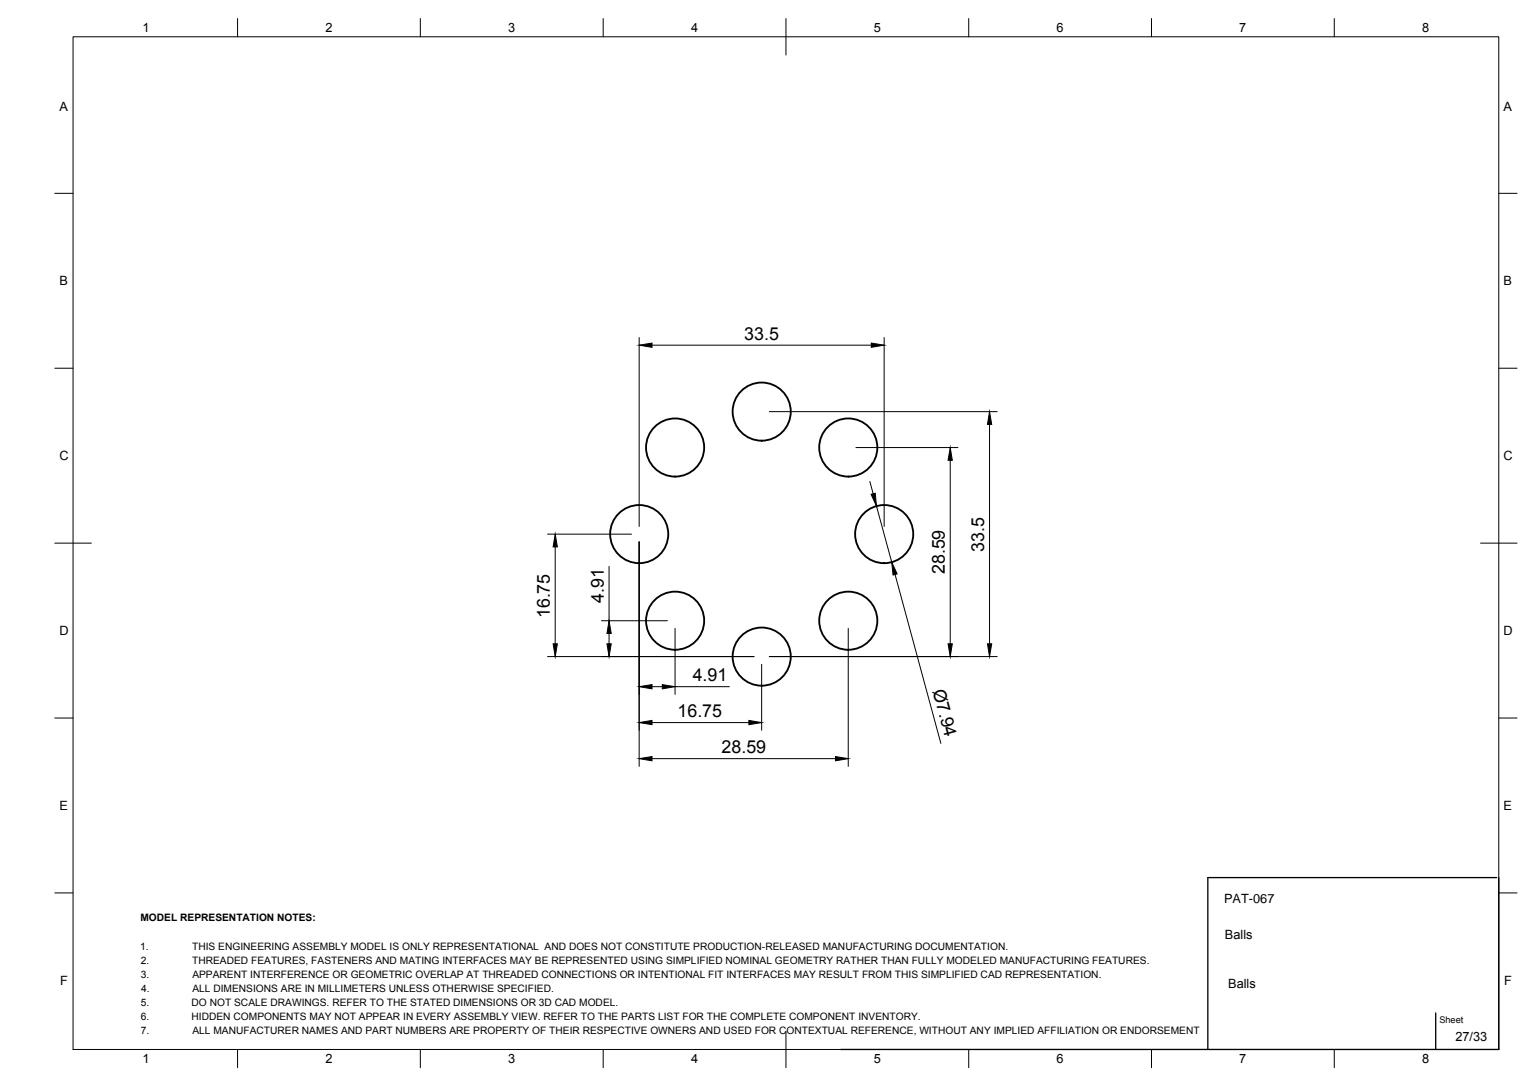
ISO-10303-21;
HEADER;
/* Generated by software containing ST-Developer
 * from STEP Tools, Inc. (www.steptools.com) 
 */

FILE_DESCRIPTION(
/* description */ ('Lifting hook block with sheave'),
/* implementation_level */ '2;1');

FILE_NAME(
/* name */ 'Balls.step',
/* time_stamp */ '2026-10-28T03:23:54-07:00',
/* author */ (''),
/* organization */ (''),
/* preprocessor_version */ 'ST-DEVELOPER v20.2',
/* originating_system */ 'Autodesk Translation Framework v15.17.0.0',
/* authorisation */ '');

FILE_SCHEMA (('AUTOMOTIVE_DESIGN { 1 0 10303 214 3 1 1 }'));
ENDSEC;

DATA;
#10=MECHANICAL_DESIGN_GEOMETRIC_PRESENTATION_REPRESENTATION('',(#373,#374,#375,#376,#377,#378,#379,#380),#9391);
#29=SPHERICAL_SURFACE('',#5724,0.3969);
#30=SPHERICAL_SURFACE('',#5726,0.3969);
#31=SPHERICAL_SURFACE('',#5728,0.3969);
#32=SPHERICAL_SURFACE('',#5730,0.3969);
#33=SPHERICAL_SURFACE('',#5732,0.3969);
#34=SPHERICAL_SURFACE('',#5734,0.3969);
#35=SPHERICAL_SURFACE('',#5736,0.3969);
#36=SPHERICAL_SURFACE('',#5738,0.3969);
#313=SHAPE_REPRESENTATION_RELATIONSHIP('SRR','None',#9546,#343);
#343=ADVANCED_BREP_SHAPE_REPRESENTATION('',(#409,#410,#411,#412,#413,#414,
#415,#416),#9381);
#373=STYLED_ITEM('',(#9759),#409);
#374=STYLED_ITEM('',(#9759),#410);
#375=STYLED_ITEM('',(#9759),#411);
#376=STYLED_ITEM('',(#9759),#412);
#377=STYLED_ITEM('',(#9759),#413);
#378=STYLED_ITEM('',(#9759),#414);
#379=STYLED_ITEM('',(#9759),#415);
#380=STYLED_ITEM('',(#9759),#416);
#409=MANIFOLD_SOLID_BREP('Body1',#4911);
#410=MANIFOLD_SOLID_BREP('Body2',#4912);
#411=MANIFOLD_SOLID_BREP('Body3',#4913);
#412=MANIFOLD_SOLID_BREP('Body4',#4914);
#413=MANIFOLD_SOLID_BREP('Body5',#4915);
#414=MANIFOLD_SOLID_BREP('Body6',#4916);
#415=MANIFOLD_SOLID_BREP('Body7',#4917);
#416=MANIFOLD_SOLID_BREP('Body8',#4918);
#1425=FACE_OUTER_BOUND('',#1813,.T.);
#1426=FACE_OUTER_BOUND('',#1814,.T.);
#1427=FACE_OUTER_BOUND('',#1815,.T.);
#1428=FACE_OUTER_BOUND('',#1816,.T.);
#1429=FACE_OUTER_BOUND('',#1817,.T.);
#1430=FACE_OUTER_BOUND('',#1818,.T.);
#1431=FACE_OUTER_BOUND('',#1819,.T.);
#1432=FACE_OUTER_BOUND('',#1820,.T.);
#1813=EDGE_LOOP('',(#4098,#4099));
#1814=EDGE_LOOP('',(#4100,#4101));
#1815=EDGE_LOOP('',(#4102,#4103));
#1816=EDGE_LOOP('',(#4104,#4105));
#1817=EDGE_LOOP('',(#4106,#4107));
#1818=EDGE_LOOP('',(#4108,#4109));
#1819=EDGE_LOOP('',(#4110,#4111));
#1820=EDGE_LOOP('',(#4112,#4113));
#2125=CIRCLE('',#5725,0.3969);
#2126=CIRCLE('',#5727,0.3969);
#2127=CIRCLE('',#5729,0.3969);
#2128=CIRCLE('',#5731,0.3969);
#2129=CIRCLE('',#5733,0.3969);
#2130=CIRCLE('',#5735,0.3969);
#2131=CIRCLE('',#5737,0.3969);
#2132=CIRCLE('',#5739,0.3969);
#2492=VERTEX_POINT('',#8555);
#2493=VERTEX_POINT('',#8556);
#2494=VERTEX_POINT('',#8559);
#2495=VERTEX_POINT('',#8560);
#2496=VERTEX_POINT('',#8563);
#2497=VERTEX_POINT('',#8564);
#2498=VERTEX_POINT('',#8567);
#2499=VERTEX_POINT('',#8568);
#2500=VERTEX_POINT('',#8571);
#2501=VERTEX_POINT('',#8572);
#2502=VERTEX_POINT('',#8575);
#2503=VERTEX_POINT('',#8576);
#2504=VERTEX_POINT('',#8579);
#2505=VERTEX_POINT('',#8580);
#2506=VERTEX_POINT('',#8583);
#2507=VERTEX_POINT('',#8584);
#3053=EDGE_CURVE('',#2492,#2493,#2125,.T.);
#3054=EDGE_CURVE('',#2494,#2495,#2126,.T.);
#3055=EDGE_CURVE('',#2496,#2497,#2127,.T.);
#3056=EDGE_CURVE('',#2498,#2499,#2128,.T.);
#3057=EDGE_CURVE('',#2500,#2501,#2129,.T.);
#3058=EDGE_CURVE('',#2502,#2503,#2130,.T.);
#3059=EDGE_CURVE('',#2504,#2505,#2131,.T.);
#3060=EDGE_CURVE('',#2506,#2507,#2132,.T.);
#4098=ORIENTED_EDGE('',*,*,#3053,.T.);
#4099=ORIENTED_EDGE('',*,*,#3053,.F.);
#4100=ORIENTED_EDGE('',*,*,#3054,.T.);
#4101=ORIENTED_EDGE('',*,*,#3054,.F.);
#4102=ORIENTED_EDGE('',*,*,#3055,.T.);
#4103=ORIENTED_EDGE('',*,*,#3055,.F.);
#4104=ORIENTED_EDGE('',*,*,#3056,.T.);
#4105=ORIENTED_EDGE('',*,*,#3056,.F.);
#4106=ORIENTED_EDGE('',*,*,#3057,.T.);
#4107=ORIENTED_EDGE('',*,*,#3057,.F.);
#4108=ORIENTED_EDGE('',*,*,#3058,.T.);
#4109=ORIENTED_EDGE('',*,*,#3058,.F.);
#4110=ORIENTED_EDGE('',*,*,#3059,.T.);
#4111=ORIENTED_EDGE('',*,*,#3059,.F.);
#4112=ORIENTED_EDGE('',*,*,#3060,.T.);
#4113=ORIENTED_EDGE('',*,*,#3060,.F.);
#4801=ADVANCED_FACE('',(#1425),#29,.T.);
#4802=ADVANCED_FACE('',(#1426),#30,.T.);
#4803=ADVANCED_FACE('',(#1427),#31,.T.);
#4804=ADVANCED_FACE('',(#1428),#32,.T.);
#4805=ADVANCED_FACE('',(#1429),#33,.T.);
#4806=ADVANCED_FACE('',(#1430),#34,.T.);
#4807=ADVANCED_FACE('',(#1431),#35,.T.);
#4808=ADVANCED_FACE('',(#1432),#36,.T.);
#4911=CLOSED_SHELL('',(#4801));
#4912=CLOSED_SHELL('',(#4802));
#4913=CLOSED_SHELL('',(#4803));
#4914=CLOSED_SHELL('',(#4804));
#4915=CLOSED_SHELL('',(#4805));
#4916=CLOSED_SHELL('',(#4806));
#4917=CLOSED_SHELL('',(#4807));
#4918=CLOSED_SHELL('',(#4808));
#5723=AXIS2_PLACEMENT_3D('',#8553,#7069,#7070);
#5724=AXIS2_PLACEMENT_3D('',#8554,#7071,#7072);
#5725=AXIS2_PLACEMENT_3D('',#8557,#7073,#7074);
#5726=AXIS2_PLACEMENT_3D('',#8558,#7075,#7076);
#5727=AXIS2_PLACEMENT_3D('',#8561,#7077,#7078);
#5728=AXIS2_PLACEMENT_3D('',#8562,#7079,#7080);
#5729=AXIS2_PLACEMENT_3D('',#8565,#7081,#7082);
#5730=AXIS2_PLACEMENT_3D('',#8566,#7083,#7084);
#5731=AXIS2_PLACEMENT_3D('',#8569,#7085,#7086);
#5732=AXIS2_PLACEMENT_3D('',#8570,#7087,#7088);
#5733=AXIS2_PLACEMENT_3D('',#8573,#7089,#7090);
#5734=AXIS2_PLACEMENT_3D('',#8574,#7091,#7092);
#5735=AXIS2_PLACEMENT_3D('',#8577,#7093,#7094);
#5736=AXIS2_PLACEMENT_3D('',#8578,#7095,#7096);
#5737=AXIS2_PLACEMENT_3D('',#8581,#7097,#7098);
#5738=AXIS2_PLACEMENT_3D('',#8582,#7099,#7100);
#5739=AXIS2_PLACEMENT_3D('',#8585,#7101,#7102);
#7069=DIRECTION('axis',(0.,0.,1.));
#7070=DIRECTION('refdir',(1.,0.,0.));
#7071=DIRECTION('center_axis',(0.,0.,1.));
#7072=DIRECTION('ref_axis',(1.,0.,0.));
#7073=DIRECTION('center_axis',(1.22464679914735E-16,-1.,0.));
#7074=DIRECTION('ref_axis',(-1.,-1.22464679914735E-16,0.));
#7075=DIRECTION('center_axis',(0.707106781186548,0.,0.707106781186548));
#7076=DIRECTION('ref_axis',(0.707106781186548,0.,-0.707106781186548));
#7077=DIRECTION('center_axis',(8.65956056235493E-17,-1.,-8.65956056235493E-17));
#7078=DIRECTION('ref_axis',(-0.707106781186548,-1.22464679914735E-16,0.707106781186548));
#7079=DIRECTION('center_axis',(1.,0.,0.));
#7080=DIRECTION('ref_axis',(6.12323399573677E-17,0.,-1.));
#7081=DIRECTION('center_axis',(7.49879891330929E-33,-1.,-1.22464679914735E-16));
#7082=DIRECTION('ref_axis',(-6.12323399573677E-17,-1.22464679914735E-16,
1.));
#7083=DIRECTION('center_axis',(0.707106781186548,0.,-0.707106781186548));
#7084=DIRECTION('ref_axis',(-0.707106781186548,0.,-0.707106781186548));
#7085=DIRECTION('center_axis',(-8.65956056235493E-17,-1.,-8.65956056235493E-17));
#7086=DIRECTION('ref_axis',(0.707106781186548,-1.22464679914735E-16,0.707106781186548));
#7087=DIRECTION('center_axis',(0.,0.,-1.));
#7088=DIRECTION('ref_axis',(-1.,0.,-1.22464679914735E-16));
#7089=DIRECTION('center_axis',(-1.22464679914735E-16,-1.,-1.49975978266186E-32));
#7090=DIRECTION('ref_axis',(1.,-1.22464679914735E-16,1.22464679914735E-16));
#7091=DIRECTION('center_axis',(-0.707106781186548,0.,-0.707106781186548));
#7092=DIRECTION('ref_axis',(-0.707106781186548,0.,0.707106781186548));
#7093=DIRECTION('center_axis',(-8.65956056235493E-17,-1.,8.65956056235493E-17));
#7094=DIRECTION('ref_axis',(0.707106781186548,-1.22464679914735E-16,-0.707106781186548));
#7095=DIRECTION('center_axis',(-1.,0.,0.));
#7096=DIRECTION('ref_axis',(-1.83697019872103E-16,0.,1.));
#7097=DIRECTION('center_axis',(-2.24963967399279E-32,-1.,1.22464679914735E-16));
#7098=DIRECTION('ref_axis',(1.83697019872103E-16,-1.22464679914735E-16,
-1.));
#7099=DIRECTION('center_axis',(-0.707106781186548,0.,0.707106781186548));
#7100=DIRECTION('ref_axis',(0.707106781186548,0.,0.707106781186548));
#7101=DIRECTION('center_axis',(8.65956056235493E-17,-1.,8.65956056235494E-17));
#7102=DIRECTION('ref_axis',(-0.707106781186548,-1.22464679914735E-16,-0.707106781186548));
#8553=CARTESIAN_POINT('',(0.,0.,0.));
#8554=CARTESIAN_POINT('Origin',(1.675,0.,0.));
#8555=CARTESIAN_POINT('',(1.675,-2.97627328869245E-33,0.3969));
#8556=CARTESIAN_POINT('',(1.675,-2.97627328869245E-33,-0.3969));
#8557=CARTESIAN_POINT('Origin',(1.675,0.,0.));
#8558=CARTESIAN_POINT('Origin',(1.18440385848747,0.,-1.18440385848747));
#8559=CARTESIAN_POINT('',(1.46505453994041,3.1867025333467E-33,-0.903753177034526));
#8560=CARTESIAN_POINT('',(0.903753177034527,-9.13924911073161E-33,-1.46505453994041));
#8561=CARTESIAN_POINT('Origin',(1.18440385848747,0.,-1.18440385848747));
#8562=CARTESIAN_POINT('Origin',(1.02564169428591E-16,0.,-1.675));
#8563=CARTESIAN_POINT('',(0.3969,-2.97627328869246E-33,-1.675));
#8564=CARTESIAN_POINT('',(-0.3969,-2.97627328869245E-33,-1.675));
#8565=CARTESIAN_POINT('Origin',(1.02564169428591E-16,0.,-1.675));
#8566=CARTESIAN_POINT('Origin',(-1.18440385848747,0.,-1.18440385848747));
#8567=CARTESIAN_POINT('',(-0.903753177034526,3.1867025333467E-33,-1.46505453994041));
#8568=CARTESIAN_POINT('',(-1.46505453994041,-9.13924911073161E-33,-0.903753177034527));
#8569=CARTESIAN_POINT('Origin',(-1.18440385848747,0.,-1.18440385848747));
#8570=CARTESIAN_POINT('Origin',(-1.675,0.,-2.05128338857182E-16));
#8571=CARTESIAN_POINT('',(-1.675,-2.97627328869246E-33,-0.3969));
#8572=CARTESIAN_POINT('',(-1.675,-2.97627328869245E-33,0.3969));
#8573=CARTESIAN_POINT('Origin',(-1.675,0.,-2.05128338857182E-16));
#8574=CARTESIAN_POINT('Origin',(-1.18440385848747,0.,1.18440385848747));
#8575=CARTESIAN_POINT('',(-1.46505453994041,6.26819044436628E-33,0.903753177034526));
#8576=CARTESIAN_POINT('',(-0.903753177034527,-1.22207370217512E-32,1.46505453994041));
#8577=CARTESIAN_POINT('Origin',(-1.18440385848747,0.,1.18440385848747));
#8578=CARTESIAN_POINT('Origin',(-3.07692508285772E-16,0.,1.675));
#8579=CARTESIAN_POINT('',(-0.3969,-2.97627328869246E-33,1.675));
#8580=CARTESIAN_POINT('',(0.396899999999999,-2.97627328869245E-33,1.675));
#8581=CARTESIAN_POINT('Origin',(-3.07692508285772E-16,0.,1.675));
#8582=CARTESIAN_POINT('Origin',(1.18440385848747,0.,1.18440385848747));
#8583=CARTESIAN_POINT('',(0.903753177034526,9.34967835538585E-33,1.46505453994041));
#8584=CARTESIAN_POINT('',(1.46505453994041,-1.53022249327708E-32,0.903753177034527));
#8585=CARTESIAN_POINT('Origin',(1.18440385848747,0.,1.18440385848747));
#9344=UNCERTAINTY_MEASURE_WITH_UNIT(LENGTH_MEASURE(0.001),#9392,
'DISTANCE_ACCURACY_VALUE',
'Maximum model space distance between geometric entities at asserted c
onnectivities');
#9354=UNCERTAINTY_MEASURE_WITH_UNIT(LENGTH_MEASURE(0.001),#9392,
'DISTANCE_ACCURACY_VALUE',
'Maximum model space distance between geometric entities at asserted c
onnectivities');
#9381=(
GEOMETRIC_REPRESENTATION_CONTEXT(3)
GLOBAL_UNCERTAINTY_ASSIGNED_CONTEXT((#9344))
GLOBAL_UNIT_ASSIGNED_CONTEXT((#9392,#9394,#9395))
REPRESENTATION_CONTEXT('','3D')
);
#9391=(
GEOMETRIC_REPRESENTATION_CONTEXT(3)
GLOBAL_UNCERTAINTY_ASSIGNED_CONTEXT((#9354))
GLOBAL_UNIT_ASSIGNED_CONTEXT((#9392,#9394,#9395))
REPRESENTATION_CONTEXT('','3D')
);
#9392=(
LENGTH_UNIT()
NAMED_UNIT(*)
SI_UNIT(.CENTI.,.METRE.)
);
#9394=(
NAMED_UNIT(*)
PLANE_ANGLE_UNIT()
SI_UNIT($,.RADIAN.)
);
#9395=(
NAMED_UNIT(*)
SI_UNIT($,.STERADIAN.)
SOLID_ANGLE_UNIT()
);
#9422=SHAPE_DEFINITION_REPRESENTATION(#9483,#9546);
#9483=PRODUCT_DEFINITION_SHAPE('',$,#9583);
#9546=SHAPE_REPRESENTATION('',(#5723),#9381);
#9556=PRODUCT_DEFINITION_CONTEXT('part definition',#9666,'design');
#9583=PRODUCT_DEFINITION('Balls','Balls',#9619,#9556);
#9619=PRODUCT_DEFINITION_FORMATION('',$,#9694);
#9666=APPLICATION_CONTEXT(
'Core Data for Automotive Mechanical Design Process');
#9667=PRODUCT_CONTEXT('part definition',#9666,'mechanical');
#9694=PRODUCT('Balls','Balls','Balls',(#9667));
#9753=COLOUR_RGB('Grey',0.48,0.52,0.57);
#9754=FILL_AREA_STYLE_COLOUR('',#9753);
#9755=FILL_AREA_STYLE('',(#9754));
#9756=SURFACE_STYLE_FILL_AREA(#9755);
#9757=SURFACE_SIDE_STYLE('',(#9756));
#9758=SURFACE_STYLE_USAGE(.BOTH.,#9757);
#9759=PRESENTATION_STYLE_ASSIGNMENT((#9758));
ENDSEC;
END-ISO-10303-21;
